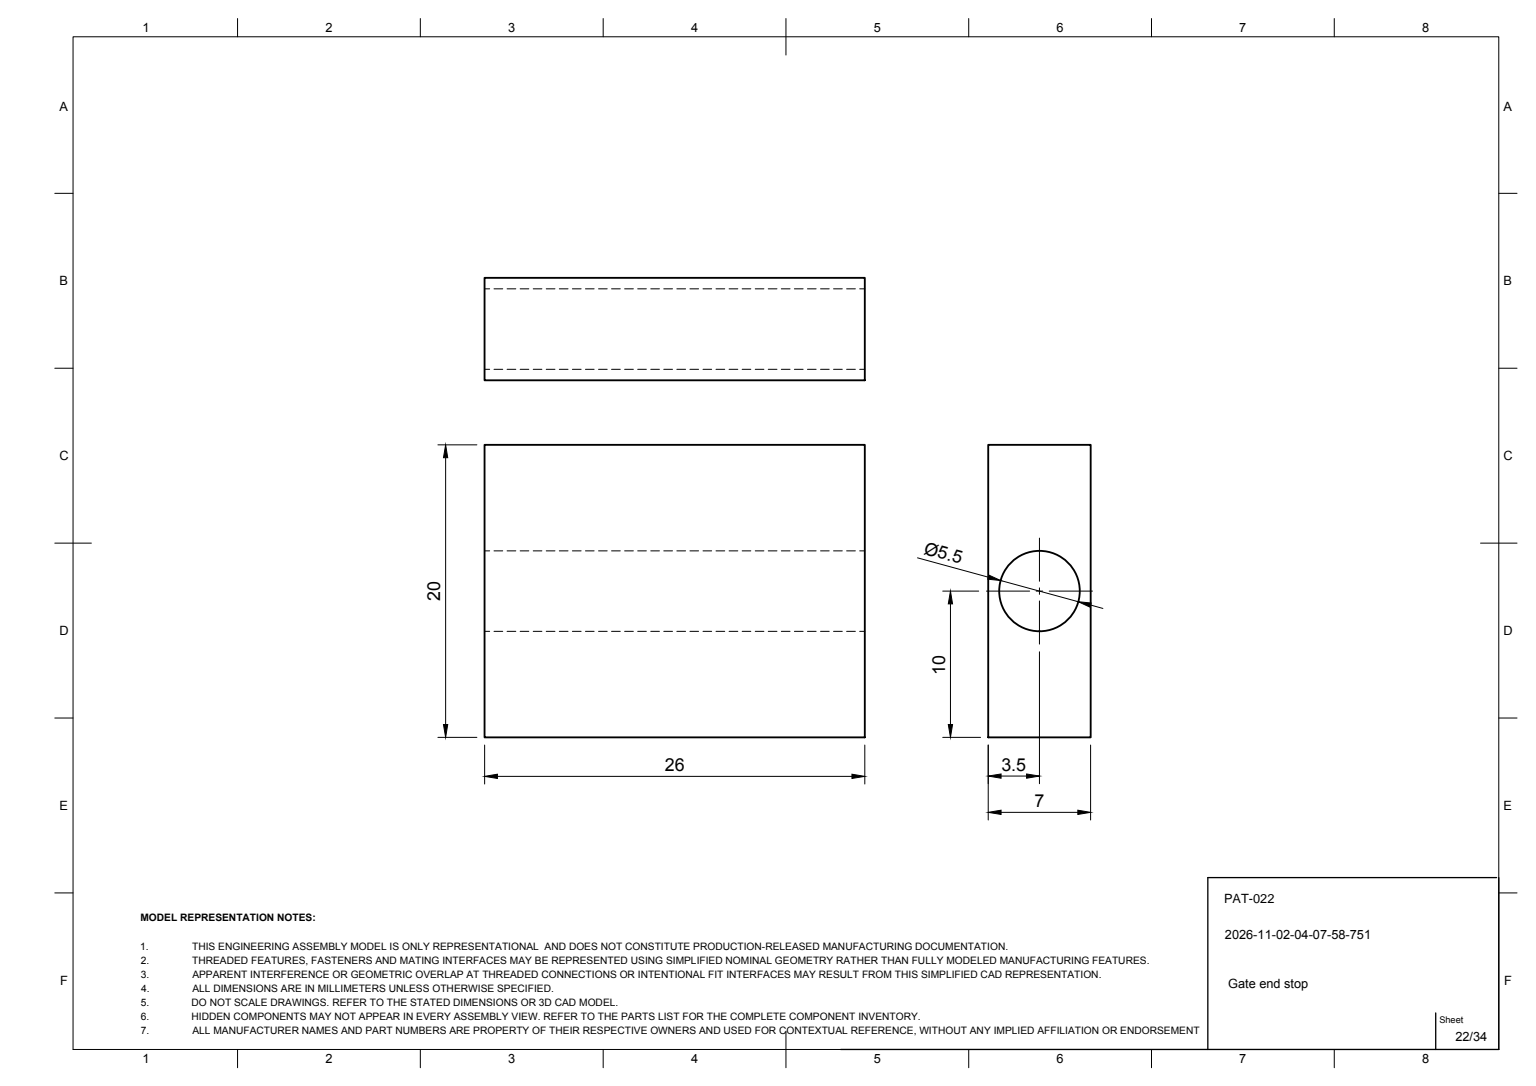
ISO-10303-21;
HEADER;
/* Generated by software containing ST-Developer
 * from STEP Tools, Inc. (www.steptools.com) 
 */

FILE_DESCRIPTION(
/* description */ ('Chute with adjustable gate'),
/* implementation_level */ '2;1');

FILE_NAME(
/* name */ 'Gate end stop.step',
/* time_stamp */ '2026-10-27T10:52:28-07:00',
/* author */ (''),
/* organization */ (''),
/* preprocessor_version */ 'ST-DEVELOPER v20.2',
/* originating_system */ 'Autodesk Translation Framework v15.17.0.0',
/* authorisation */ '');

FILE_SCHEMA (('AUTOMOTIVE_DESIGN { 1 0 10303 214 3 1 1 }'));
ENDSEC;

DATA;
#10=MECHANICAL_DESIGN_GEOMETRIC_PRESENTATION_REPRESENTATION('',(#431),#13094);
#367=SHAPE_REPRESENTATION_RELATIONSHIP('SRR','None',#13268,#399);
#399=ADVANCED_BREP_SHAPE_REPRESENTATION('',(#463),#13077);
#431=STYLED_ITEM('',(#13481),#463);
#463=MANIFOLD_SOLID_BREP('Body1',#7614);
#546=FACE_BOUND('',#1574,.T.);
#547=FACE_BOUND('',#1577,.T.);
#722=PLANE('',#8255);
#723=PLANE('',#8256);
#724=PLANE('',#8257);
#725=PLANE('',#8258);
#726=PLANE('',#8259);
#727=PLANE('',#8260);
#1084=FACE_OUTER_BOUND('',#1571,.T.);
#1085=FACE_OUTER_BOUND('',#1572,.T.);
#1086=FACE_OUTER_BOUND('',#1573,.T.);
#1087=FACE_OUTER_BOUND('',#1575,.T.);
#1088=FACE_OUTER_BOUND('',#1576,.T.);
#1089=FACE_OUTER_BOUND('',#1578,.T.);
#1090=FACE_OUTER_BOUND('',#1579,.T.);
#1571=EDGE_LOOP('',(#5942,#5943,#5944,#5945));
#1572=EDGE_LOOP('',(#5946,#5947,#5948,#5949));
#1573=EDGE_LOOP('',(#5950,#5951,#5952,#5953));
#1574=EDGE_LOOP('',(#5954));
#1575=EDGE_LOOP('',(#5955,#5956,#5957,#5958));
#1576=EDGE_LOOP('',(#5959,#5960,#5961,#5962));
#1577=EDGE_LOOP('',(#5963));
#1578=EDGE_LOOP('',(#5964,#5965,#5966,#5967));
#1579=EDGE_LOOP('',(#5968,#5969,#5970,#5971));
#2162=LINE('',#11723,#2939);
#2163=LINE('',#11728,#2940);
#2164=LINE('',#11730,#2941);
#2165=LINE('',#11732,#2942);
#2166=LINE('',#11733,#2943);
#2167=LINE('',#11736,#2944);
#2168=LINE('',#11738,#2945);
#2169=LINE('',#11739,#2946);
#2170=LINE('',#11742,#2947);
#2171=LINE('',#11744,#2948);
#2172=LINE('',#11745,#2949);
#2173=LINE('',#11747,#2950);
#2174=LINE('',#11748,#2951);
#2939=VECTOR('',#9536,0.275);
#2940=VECTOR('',#9541,1.);
#2941=VECTOR('',#9542,1.);
#2942=VECTOR('',#9543,1.);
#2943=VECTOR('',#9544,1.);
#2944=VECTOR('',#9547,1.);
#2945=VECTOR('',#9548,1.);
#2946=VECTOR('',#9549,1.);
#2947=VECTOR('',#9552,1.);
#2948=VECTOR('',#9553,1.);
#2949=VECTOR('',#9554,1.);
#2950=VECTOR('',#9557,1.);
#2951=VECTOR('',#9558,1.);
#3490=CIRCLE('',#8253,0.275);
#3491=CIRCLE('',#8254,0.275);
#3845=VERTEX_POINT('',#11720);
#3846=VERTEX_POINT('',#11722);
#3847=VERTEX_POINT('',#11726);
#3848=VERTEX_POINT('',#11727);
#3849=VERTEX_POINT('',#11729);
#3850=VERTEX_POINT('',#11731);
#3851=VERTEX_POINT('',#11735);
#3852=VERTEX_POINT('',#11737);
#3853=VERTEX_POINT('',#11741);
#3854=VERTEX_POINT('',#11743);
#4604=EDGE_CURVE('',#3845,#3845,#3490,.T.);
#4605=EDGE_CURVE('',#3845,#3846,#2162,.T.);
#4606=EDGE_CURVE('',#3846,#3846,#3491,.T.);
#4607=EDGE_CURVE('',#3847,#3848,#2163,.T.);
#4608=EDGE_CURVE('',#3848,#3849,#2164,.T.);
#4609=EDGE_CURVE('',#3850,#3849,#2165,.T.);
#4610=EDGE_CURVE('',#3847,#3850,#2166,.T.);
#4611=EDGE_CURVE('',#3851,#3847,#2167,.T.);
#4612=EDGE_CURVE('',#3852,#3850,#2168,.T.);
#4613=EDGE_CURVE('',#3851,#3852,#2169,.T.);
#4614=EDGE_CURVE('',#3853,#3851,#2170,.T.);
#4615=EDGE_CURVE('',#3854,#3852,#2171,.T.);
#4616=EDGE_CURVE('',#3853,#3854,#2172,.T.);
#4617=EDGE_CURVE('',#3848,#3853,#2173,.T.);
#4618=EDGE_CURVE('',#3849,#3854,#2174,.T.);
#5942=ORIENTED_EDGE('',*,*,#4604,.F.);
#5943=ORIENTED_EDGE('',*,*,#4605,.T.);
#5944=ORIENTED_EDGE('',*,*,#4606,.F.);
#5945=ORIENTED_EDGE('',*,*,#4605,.F.);
#5946=ORIENTED_EDGE('',*,*,#4607,.T.);
#5947=ORIENTED_EDGE('',*,*,#4608,.T.);
#5948=ORIENTED_EDGE('',*,*,#4609,.F.);
#5949=ORIENTED_EDGE('',*,*,#4610,.F.);
#5950=ORIENTED_EDGE('',*,*,#4611,.T.);
#5951=ORIENTED_EDGE('',*,*,#4610,.T.);
#5952=ORIENTED_EDGE('',*,*,#4612,.F.);
#5953=ORIENTED_EDGE('',*,*,#4613,.F.);
#5954=ORIENTED_EDGE('',*,*,#4606,.T.);
#5955=ORIENTED_EDGE('',*,*,#4614,.T.);
#5956=ORIENTED_EDGE('',*,*,#4613,.T.);
#5957=ORIENTED_EDGE('',*,*,#4615,.F.);
#5958=ORIENTED_EDGE('',*,*,#4616,.F.);
#5959=ORIENTED_EDGE('',*,*,#4617,.T.);
#5960=ORIENTED_EDGE('',*,*,#4616,.T.);
#5961=ORIENTED_EDGE('',*,*,#4618,.F.);
#5962=ORIENTED_EDGE('',*,*,#4608,.F.);
#5963=ORIENTED_EDGE('',*,*,#4604,.T.);
#5964=ORIENTED_EDGE('',*,*,#4618,.T.);
#5965=ORIENTED_EDGE('',*,*,#4615,.T.);
#5966=ORIENTED_EDGE('',*,*,#4612,.T.);
#5967=ORIENTED_EDGE('',*,*,#4609,.T.);
#5968=ORIENTED_EDGE('',*,*,#4617,.F.);
#5969=ORIENTED_EDGE('',*,*,#4607,.F.);
#5970=ORIENTED_EDGE('',*,*,#4611,.F.);
#5971=ORIENTED_EDGE('',*,*,#4614,.F.);
#7144=CYLINDRICAL_SURFACE('',#8252,0.275);
#7352=ADVANCED_FACE('',(#1084),#7144,.F.);
#7353=ADVANCED_FACE('',(#1085),#722,.T.);
#7354=ADVANCED_FACE('',(#1086,#546),#723,.T.);
#7355=ADVANCED_FACE('',(#1087),#724,.T.);
#7356=ADVANCED_FACE('',(#1088,#547),#725,.T.);
#7357=ADVANCED_FACE('',(#1089),#726,.T.);
#7358=ADVANCED_FACE('',(#1090),#727,.F.);
#7614=CLOSED_SHELL('',(#7352,#7353,#7354,#7355,#7356,#7357,#7358));
#8251=AXIS2_PLACEMENT_3D('',#11718,#9530,#9531);
#8252=AXIS2_PLACEMENT_3D('',#11719,#9532,#9533);
#8253=AXIS2_PLACEMENT_3D('',#11721,#9534,#9535);
#8254=AXIS2_PLACEMENT_3D('',#11724,#9537,#9538);
#8255=AXIS2_PLACEMENT_3D('',#11725,#9539,#9540);
#8256=AXIS2_PLACEMENT_3D('',#11734,#9545,#9546);
#8257=AXIS2_PLACEMENT_3D('',#11740,#9550,#9551);
#8258=AXIS2_PLACEMENT_3D('',#11746,#9555,#9556);
#8259=AXIS2_PLACEMENT_3D('',#11749,#9559,#9560);
#8260=AXIS2_PLACEMENT_3D('',#11750,#9561,#9562);
#9530=DIRECTION('axis',(0.,0.,1.));
#9531=DIRECTION('refdir',(1.,0.,0.));
#9532=DIRECTION('center_axis',(1.,0.,0.));
#9533=DIRECTION('ref_axis',(0.,0.,-1.));
#9534=DIRECTION('center_axis',(1.,0.,0.));
#9535=DIRECTION('ref_axis',(0.,0.,-1.));
#9536=DIRECTION('',(1.,0.,0.));
#9537=DIRECTION('center_axis',(-1.,0.,0.));
#9538=DIRECTION('ref_axis',(0.,0.,-1.));
#9539=DIRECTION('center_axis',(0.,1.,0.));
#9540=DIRECTION('ref_axis',(-1.,0.,0.));
#9541=DIRECTION('',(-1.,0.,0.));
#9542=DIRECTION('',(0.,0.,1.));
#9543=DIRECTION('',(-1.,0.,0.));
#9544=DIRECTION('',(0.,0.,1.));
#9545=DIRECTION('center_axis',(1.,0.,0.));
#9546=DIRECTION('ref_axis',(0.,1.,0.));
#9547=DIRECTION('',(0.,1.,0.));
#9548=DIRECTION('',(0.,1.,0.));
#9549=DIRECTION('',(0.,0.,1.));
#9550=DIRECTION('center_axis',(0.,-1.,0.));
#9551=DIRECTION('ref_axis',(1.,0.,0.));
#9552=DIRECTION('',(1.,0.,0.));
#9553=DIRECTION('',(1.,0.,0.));
#9554=DIRECTION('',(0.,0.,1.));
#9555=DIRECTION('center_axis',(-1.,0.,0.));
#9556=DIRECTION('ref_axis',(0.,-1.,0.));
#9557=DIRECTION('',(0.,-1.,0.));
#9558=DIRECTION('',(0.,-1.,0.));
#9559=DIRECTION('center_axis',(0.,0.,1.));
#9560=DIRECTION('ref_axis',(1.,0.,0.));
#9561=DIRECTION('center_axis',(0.,0.,1.));
#9562=DIRECTION('ref_axis',(1.,0.,0.));
#11718=CARTESIAN_POINT('',(0.,0.,0.));
#11719=CARTESIAN_POINT('Origin',(-1.5,11.,6.95));
#11720=CARTESIAN_POINT('',(-1.4,11.,7.225));
#11721=CARTESIAN_POINT('Origin',(-1.4,11.,6.95));
#11722=CARTESIAN_POINT('',(1.2,11.,7.225));
#11723=CARTESIAN_POINT('',(-1.5,11.,7.225));
#11724=CARTESIAN_POINT('Origin',(1.2,11.,6.95));
#11725=CARTESIAN_POINT('Origin',(1.2,12.,6.6));
#11726=CARTESIAN_POINT('',(1.2,12.,6.6));
#11727=CARTESIAN_POINT('',(-1.4,12.,6.6));
#11728=CARTESIAN_POINT('',(1.2,12.,6.6));
#11729=CARTESIAN_POINT('',(-1.4,12.,7.3));
#11730=CARTESIAN_POINT('',(-1.4,12.,6.6));
#11731=CARTESIAN_POINT('',(1.2,12.,7.3));
#11732=CARTESIAN_POINT('',(1.2,12.,7.3));
#11733=CARTESIAN_POINT('',(1.2,12.,6.6));
#11734=CARTESIAN_POINT('Origin',(1.2,10.,6.6));
#11735=CARTESIAN_POINT('',(1.2,10.,6.6));
#11736=CARTESIAN_POINT('',(1.2,10.,6.6));
#11737=CARTESIAN_POINT('',(1.2,10.,7.3));
#11738=CARTESIAN_POINT('',(1.2,10.,7.3));
#11739=CARTESIAN_POINT('',(1.2,10.,6.6));
#11740=CARTESIAN_POINT('Origin',(-1.4,10.,6.6));
#11741=CARTESIAN_POINT('',(-1.4,10.,6.6));
#11742=CARTESIAN_POINT('',(-1.4,10.,6.6));
#11743=CARTESIAN_POINT('',(-1.4,10.,7.3));
#11744=CARTESIAN_POINT('',(-1.4,10.,7.3));
#11745=CARTESIAN_POINT('',(-1.4,10.,6.6));
#11746=CARTESIAN_POINT('Origin',(-1.4,12.,6.6));
#11747=CARTESIAN_POINT('',(-1.4,12.,6.6));
#11748=CARTESIAN_POINT('',(-1.4,12.,7.3));
#11749=CARTESIAN_POINT('Origin',(-0.1,11.,7.3));
#11750=CARTESIAN_POINT('Origin',(-0.1,11.,6.6));
#13040=UNCERTAINTY_MEASURE_WITH_UNIT(LENGTH_MEASURE(0.001),#13095,
'DISTANCE_ACCURACY_VALUE',
'Maximum model space distance between geometric entities at asserted c
onnectivities');
#13057=UNCERTAINTY_MEASURE_WITH_UNIT(LENGTH_MEASURE(0.001),#13095,
'DISTANCE_ACCURACY_VALUE',
'Maximum model space distance between geometric entities at asserted c
onnectivities');
#13077=(
GEOMETRIC_REPRESENTATION_CONTEXT(3)
GLOBAL_UNCERTAINTY_ASSIGNED_CONTEXT((#13040))
GLOBAL_UNIT_ASSIGNED_CONTEXT((#13095,#13097,#13098))
REPRESENTATION_CONTEXT('','3D')
);
#13094=(
GEOMETRIC_REPRESENTATION_CONTEXT(3)
GLOBAL_UNCERTAINTY_ASSIGNED_CONTEXT((#13057))
GLOBAL_UNIT_ASSIGNED_CONTEXT((#13095,#13097,#13098))
REPRESENTATION_CONTEXT('','3D')
);
#13095=(
LENGTH_UNIT()
NAMED_UNIT(*)
SI_UNIT(.CENTI.,.METRE.)
);
#13097=(
NAMED_UNIT(*)
PLANE_ANGLE_UNIT()
SI_UNIT($,.RADIAN.)
);
#13098=(
NAMED_UNIT(*)
SI_UNIT($,.STERADIAN.)
SOLID_ANGLE_UNIT()
);
#13118=SHAPE_DEFINITION_REPRESENTATION(#13154,#13268);
#13154=PRODUCT_DEFINITION_SHAPE('',$,#13305);
#13268=SHAPE_REPRESENTATION('',(#8251),#13077);
#13285=PRODUCT_DEFINITION_CONTEXT('part definition',#13395,'design');
#13305=PRODUCT_DEFINITION('Gate end stop','Gate end stop',#13341,#13285);
#13341=PRODUCT_DEFINITION_FORMATION('',$,#13416);
#13395=APPLICATION_CONTEXT(
'Core Data for Automotive Mechanical Design Process');
#13396=PRODUCT_CONTEXT('part definition',#13395,'mechanical');
#13416=PRODUCT('Gate end stop','Gate end stop','Gate end stop',(#13396));
#13475=COLOUR_RGB('Light Blue',0.38,0.62,0.78);
#13476=FILL_AREA_STYLE_COLOUR('',#13475);
#13477=FILL_AREA_STYLE('',(#13476));
#13478=SURFACE_STYLE_FILL_AREA(#13477);
#13479=SURFACE_SIDE_STYLE('',(#13478));
#13480=SURFACE_STYLE_USAGE(.BOTH.,#13479);
#13481=PRESENTATION_STYLE_ASSIGNMENT((#13480));
ENDSEC;
END-ISO-10303-21;
